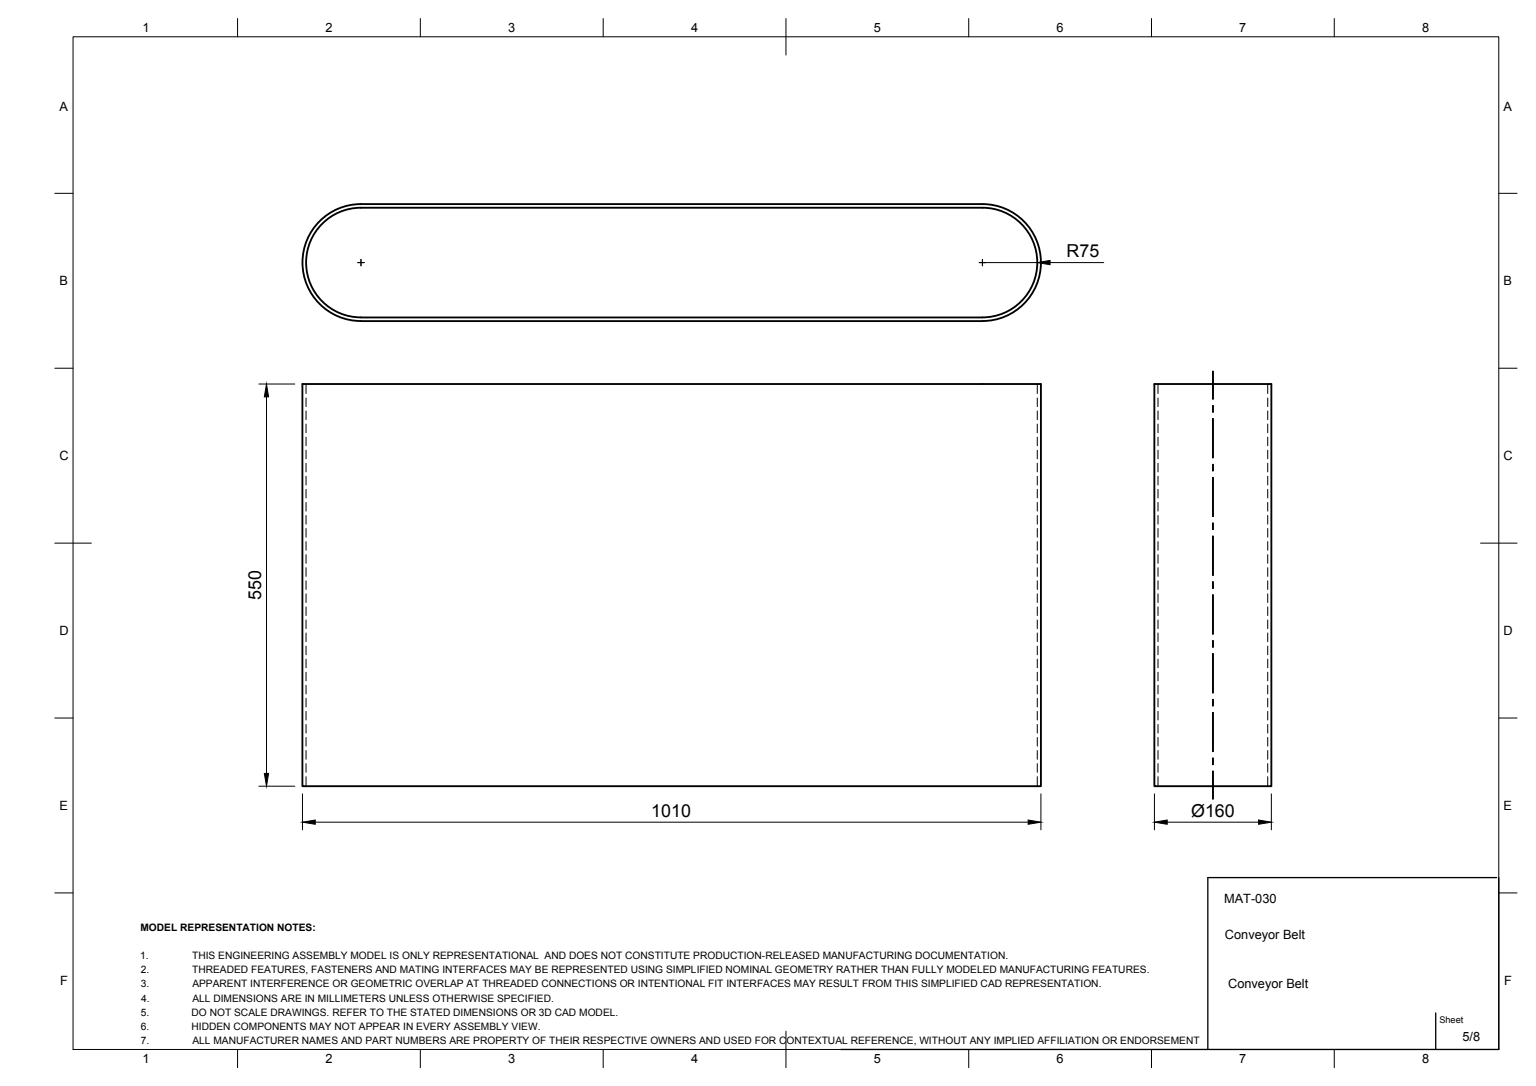
ISO-10303-21;
HEADER;
/* Generated by software containing ST-Developer
 * from STEP Tools, Inc. (www.steptools.com) 
 */

FILE_DESCRIPTION(
/* description */ ('STEP AP214'),
/* implementation_level */ '2;1');

FILE_NAME(
/* name */ 'Conveyor Belt.step',
/* time_stamp */ '2026-11-14T06:43:04-08:00',
/* author */ (''),
/* organization */ (''),
/* preprocessor_version */ 'ST-DEVELOPER v20.2',
/* originating_system */ 'Autodesk Translation Framework v15.17.0.0',
/* authorisation */ '');

FILE_SCHEMA (('AUTOMOTIVE_DESIGN { 1 0 10303 214 3 1 1 }'));
ENDSEC;

DATA;
#10=MECHANICAL_DESIGN_GEOMETRIC_PRESENTATION_REPRESENTATION('',(#198),#5658);
#176=SHAPE_REPRESENTATION_RELATIONSHIP('SRR','None',#5706,#187);
#187=ADVANCED_BREP_SHAPE_REPRESENTATION('',(#209),#5647);
#198=STYLED_ITEM('',(#5770),#209);
#209=MANIFOLD_SOLID_BREP('Body1',#3060);
#220=CYLINDRICAL_SURFACE('',#3205,80.);
#221=CYLINDRICAL_SURFACE('',#3207,80.);
#222=CYLINDRICAL_SURFACE('',#3209,75.);
#223=CYLINDRICAL_SURFACE('',#3211,75.);
#271=FACE_BOUND('',#520,.T.);
#272=FACE_BOUND('',#522,.T.);
#337=FACE_OUTER_BOUND('',#519,.T.);
#338=FACE_OUTER_BOUND('',#521,.T.);
#339=FACE_OUTER_BOUND('',#523,.T.);
#340=FACE_OUTER_BOUND('',#524,.T.);
#341=FACE_OUTER_BOUND('',#525,.T.);
#342=FACE_OUTER_BOUND('',#526,.T.);
#343=FACE_OUTER_BOUND('',#527,.T.);
#344=FACE_OUTER_BOUND('',#528,.T.);
#345=FACE_OUTER_BOUND('',#529,.T.);
#346=FACE_OUTER_BOUND('',#530,.T.);
#519=EDGE_LOOP('',(#1976,#1977,#1978,#1979));
#520=EDGE_LOOP('',(#1980,#1981,#1982,#1983));
#521=EDGE_LOOP('',(#1984,#1985,#1986,#1987));
#522=EDGE_LOOP('',(#1988,#1989,#1990,#1991));
#523=EDGE_LOOP('',(#1992,#1993,#1994,#1995));
#524=EDGE_LOOP('',(#1996,#1997,#1998,#1999));
#525=EDGE_LOOP('',(#2000,#2001,#2002,#2003));
#526=EDGE_LOOP('',(#2004,#2005,#2006,#2007));
#527=EDGE_LOOP('',(#2008,#2009,#2010,#2011));
#528=EDGE_LOOP('',(#2012,#2013,#2014,#2015));
#529=EDGE_LOOP('',(#2016,#2017,#2018,#2019));
#530=EDGE_LOOP('',(#2020,#2021,#2022,#2023));
#767=LINE('',#4494,#963);
#768=LINE('',#4497,#964);
#769=LINE('',#4500,#965);
#770=LINE('',#4504,#966);
#771=LINE('',#4511,#967);
#772=LINE('',#4514,#968);
#773=LINE('',#4519,#969);
#774=LINE('',#4522,#970);
#775=LINE('',#4524,#971);
#776=LINE('',#4525,#972);
#777=LINE('',#4527,#973);
#778=LINE('',#4529,#974);
#779=LINE('',#4532,#975);
#780=LINE('',#4533,#976);
#781=LINE('',#4535,#977);
#782=LINE('',#4537,#978);
#963=VECTOR('',#3567,1000.);
#964=VECTOR('',#3570,1000.);
#965=VECTOR('',#3571,1000.);
#966=VECTOR('',#3574,1000.);
#967=VECTOR('',#3581,1000.);
#968=VECTOR('',#3584,1000.);
#969=VECTOR('',#3587,1000.);
#970=VECTOR('',#3590,1000.);
#971=VECTOR('',#3593,1000.);
#972=VECTOR('',#3594,1000.);
#973=VECTOR('',#3597,1000.);
#974=VECTOR('',#3600,1000.);
#975=VECTOR('',#3605,1000.);
#976=VECTOR('',#3606,1000.);
#977=VECTOR('',#3609,1000.);
#978=VECTOR('',#3612,1000.);
#1159=CIRCLE('',#3196,80.);
#1160=CIRCLE('',#3197,80.);
#1161=CIRCLE('',#3198,75.);
#1162=CIRCLE('',#3199,75.);
#1163=CIRCLE('',#3201,80.);
#1164=CIRCLE('',#3202,80.);
#1165=CIRCLE('',#3203,75.);
#1166=CIRCLE('',#3204,75.);
#1314=VERTEX_POINT('',#4490);
#1315=VERTEX_POINT('',#4491);
#1316=VERTEX_POINT('',#4493);
#1317=VERTEX_POINT('',#4495);
#1318=VERTEX_POINT('',#4498);
#1319=VERTEX_POINT('',#4499);
#1320=VERTEX_POINT('',#4501);
#1321=VERTEX_POINT('',#4503);
#1322=VERTEX_POINT('',#4507);
#1323=VERTEX_POINT('',#4508);
#1324=VERTEX_POINT('',#4510);
#1325=VERTEX_POINT('',#4512);
#1326=VERTEX_POINT('',#4515);
#1327=VERTEX_POINT('',#4516);
#1328=VERTEX_POINT('',#4518);
#1329=VERTEX_POINT('',#4520);
#1571=EDGE_CURVE('',#1314,#1315,#1159,.T.);
#1572=EDGE_CURVE('',#1315,#1316,#767,.T.);
#1573=EDGE_CURVE('',#1316,#1317,#1160,.T.);
#1574=EDGE_CURVE('',#1317,#1314,#768,.T.);
#1575=EDGE_CURVE('',#1318,#1319,#769,.T.);
#1576=EDGE_CURVE('',#1320,#1318,#1161,.T.);
#1577=EDGE_CURVE('',#1321,#1320,#770,.T.);
#1578=EDGE_CURVE('',#1319,#1321,#1162,.T.);
#1579=EDGE_CURVE('',#1322,#1323,#1163,.T.);
#1580=EDGE_CURVE('',#1324,#1322,#771,.T.);
#1581=EDGE_CURVE('',#1325,#1324,#1164,.T.);
#1582=EDGE_CURVE('',#1323,#1325,#772,.T.);
#1583=EDGE_CURVE('',#1326,#1327,#1165,.T.);
#1584=EDGE_CURVE('',#1327,#1328,#773,.T.);
#1585=EDGE_CURVE('',#1328,#1329,#1166,.T.);
#1586=EDGE_CURVE('',#1329,#1326,#774,.T.);
#1587=EDGE_CURVE('',#1315,#1323,#775,.T.);
#1588=EDGE_CURVE('',#1314,#1322,#776,.T.);
#1589=EDGE_CURVE('',#1316,#1325,#777,.T.);
#1590=EDGE_CURVE('',#1317,#1324,#778,.T.);
#1591=EDGE_CURVE('',#1320,#1326,#779,.T.);
#1592=EDGE_CURVE('',#1318,#1327,#780,.T.);
#1593=EDGE_CURVE('',#1319,#1328,#781,.T.);
#1594=EDGE_CURVE('',#1321,#1329,#782,.T.);
#1976=ORIENTED_EDGE('',*,*,#1571,.T.);
#1977=ORIENTED_EDGE('',*,*,#1572,.T.);
#1978=ORIENTED_EDGE('',*,*,#1573,.T.);
#1979=ORIENTED_EDGE('',*,*,#1574,.T.);
#1980=ORIENTED_EDGE('',*,*,#1575,.F.);
#1981=ORIENTED_EDGE('',*,*,#1576,.F.);
#1982=ORIENTED_EDGE('',*,*,#1577,.F.);
#1983=ORIENTED_EDGE('',*,*,#1578,.F.);
#1984=ORIENTED_EDGE('',*,*,#1579,.F.);
#1985=ORIENTED_EDGE('',*,*,#1580,.F.);
#1986=ORIENTED_EDGE('',*,*,#1581,.F.);
#1987=ORIENTED_EDGE('',*,*,#1582,.F.);
#1988=ORIENTED_EDGE('',*,*,#1583,.T.);
#1989=ORIENTED_EDGE('',*,*,#1584,.T.);
#1990=ORIENTED_EDGE('',*,*,#1585,.T.);
#1991=ORIENTED_EDGE('',*,*,#1586,.T.);
#1992=ORIENTED_EDGE('',*,*,#1579,.T.);
#1993=ORIENTED_EDGE('',*,*,#1587,.F.);
#1994=ORIENTED_EDGE('',*,*,#1571,.F.);
#1995=ORIENTED_EDGE('',*,*,#1588,.T.);
#1996=ORIENTED_EDGE('',*,*,#1582,.T.);
#1997=ORIENTED_EDGE('',*,*,#1589,.F.);
#1998=ORIENTED_EDGE('',*,*,#1572,.F.);
#1999=ORIENTED_EDGE('',*,*,#1587,.T.);
#2000=ORIENTED_EDGE('',*,*,#1581,.T.);
#2001=ORIENTED_EDGE('',*,*,#1590,.F.);
#2002=ORIENTED_EDGE('',*,*,#1573,.F.);
#2003=ORIENTED_EDGE('',*,*,#1589,.T.);
#2004=ORIENTED_EDGE('',*,*,#1580,.T.);
#2005=ORIENTED_EDGE('',*,*,#1588,.F.);
#2006=ORIENTED_EDGE('',*,*,#1574,.F.);
#2007=ORIENTED_EDGE('',*,*,#1590,.T.);
#2008=ORIENTED_EDGE('',*,*,#1583,.F.);
#2009=ORIENTED_EDGE('',*,*,#1591,.F.);
#2010=ORIENTED_EDGE('',*,*,#1576,.T.);
#2011=ORIENTED_EDGE('',*,*,#1592,.T.);
#2012=ORIENTED_EDGE('',*,*,#1584,.F.);
#2013=ORIENTED_EDGE('',*,*,#1592,.F.);
#2014=ORIENTED_EDGE('',*,*,#1575,.T.);
#2015=ORIENTED_EDGE('',*,*,#1593,.T.);
#2016=ORIENTED_EDGE('',*,*,#1585,.F.);
#2017=ORIENTED_EDGE('',*,*,#1593,.F.);
#2018=ORIENTED_EDGE('',*,*,#1578,.T.);
#2019=ORIENTED_EDGE('',*,*,#1594,.T.);
#2020=ORIENTED_EDGE('',*,*,#1586,.F.);
#2021=ORIENTED_EDGE('',*,*,#1594,.F.);
#2022=ORIENTED_EDGE('',*,*,#1577,.T.);
#2023=ORIENTED_EDGE('',*,*,#1591,.T.);
#2786=PLANE('',#3195);
#2787=PLANE('',#3200);
#2788=PLANE('',#3206);
#2789=PLANE('',#3208);
#2790=PLANE('',#3210);
#2791=PLANE('',#3212);
#2878=ADVANCED_FACE('',(#337,#271),#2786,.T.);
#2879=ADVANCED_FACE('',(#338,#272),#2787,.F.);
#2880=ADVANCED_FACE('',(#339),#220,.T.);
#2881=ADVANCED_FACE('',(#340),#2788,.F.);
#2882=ADVANCED_FACE('',(#341),#221,.T.);
#2883=ADVANCED_FACE('',(#342),#2789,.F.);
#2884=ADVANCED_FACE('',(#343),#222,.F.);
#2885=ADVANCED_FACE('',(#344),#2790,.T.);
#2886=ADVANCED_FACE('',(#345),#223,.F.);
#2887=ADVANCED_FACE('',(#346),#2791,.T.);
#3060=CLOSED_SHELL('',(#2878,#2879,#2880,#2881,#2882,#2883,#2884,#2885,
#2886,#2887));
#3194=AXIS2_PLACEMENT_3D('',#4488,#3561,#3562);
#3195=AXIS2_PLACEMENT_3D('',#4489,#3563,#3564);
#3196=AXIS2_PLACEMENT_3D('',#4492,#3565,#3566);
#3197=AXIS2_PLACEMENT_3D('',#4496,#3568,#3569);
#3198=AXIS2_PLACEMENT_3D('',#4502,#3572,#3573);
#3199=AXIS2_PLACEMENT_3D('',#4505,#3575,#3576);
#3200=AXIS2_PLACEMENT_3D('',#4506,#3577,#3578);
#3201=AXIS2_PLACEMENT_3D('',#4509,#3579,#3580);
#3202=AXIS2_PLACEMENT_3D('',#4513,#3582,#3583);
#3203=AXIS2_PLACEMENT_3D('',#4517,#3585,#3586);
#3204=AXIS2_PLACEMENT_3D('',#4521,#3588,#3589);
#3205=AXIS2_PLACEMENT_3D('',#4523,#3591,#3592);
#3206=AXIS2_PLACEMENT_3D('',#4526,#3595,#3596);
#3207=AXIS2_PLACEMENT_3D('',#4528,#3598,#3599);
#3208=AXIS2_PLACEMENT_3D('',#4530,#3601,#3602);
#3209=AXIS2_PLACEMENT_3D('',#4531,#3603,#3604);
#3210=AXIS2_PLACEMENT_3D('',#4534,#3607,#3608);
#3211=AXIS2_PLACEMENT_3D('',#4536,#3610,#3611);
#3212=AXIS2_PLACEMENT_3D('',#4538,#3613,#3614);
#3561=DIRECTION('axis',(0.,0.,1.));
#3562=DIRECTION('refdir',(1.,0.,0.));
#3563=DIRECTION('center_axis',(1.,0.,0.));
#3564=DIRECTION('ref_axis',(0.,0.,-1.));
#3565=DIRECTION('center_axis',(1.,0.,0.));
#3566=DIRECTION('ref_axis',(0.,1.,0.));
#3567=DIRECTION('',(0.,1.,1.79594901042305E-16));
#3568=DIRECTION('center_axis',(1.,0.,0.));
#3569=DIRECTION('ref_axis',(0.,1.,0.));
#3570=DIRECTION('',(0.,-1.,-1.79594901042305E-16));
#3571=DIRECTION('',(0.,1.,1.79594901042305E-16));
#3572=DIRECTION('center_axis',(1.,0.,0.));
#3573=DIRECTION('ref_axis',(0.,0.,-1.));
#3574=DIRECTION('',(0.,-1.,-1.79594901042305E-16));
#3575=DIRECTION('center_axis',(1.,0.,0.));
#3576=DIRECTION('ref_axis',(0.,0.,-1.));
#3577=DIRECTION('center_axis',(1.,0.,0.));
#3578=DIRECTION('ref_axis',(0.,0.,-1.));
#3579=DIRECTION('center_axis',(1.,0.,0.));
#3580=DIRECTION('ref_axis',(0.,1.,0.));
#3581=DIRECTION('',(0.,-1.,-1.79594901042305E-16));
#3582=DIRECTION('center_axis',(1.,0.,0.));
#3583=DIRECTION('ref_axis',(0.,1.,0.));
#3584=DIRECTION('',(0.,1.,1.79594901042305E-16));
#3585=DIRECTION('center_axis',(1.,0.,0.));
#3586=DIRECTION('ref_axis',(0.,0.,-1.));
#3587=DIRECTION('',(0.,1.,1.79594901042305E-16));
#3588=DIRECTION('center_axis',(1.,0.,0.));
#3589=DIRECTION('ref_axis',(0.,0.,-1.));
#3590=DIRECTION('',(0.,-1.,-1.79594901042305E-16));
#3591=DIRECTION('center_axis',(-1.,0.,0.));
#3592=DIRECTION('ref_axis',(0.,0.,1.));
#3593=DIRECTION('',(-1.,0.,0.));
#3594=DIRECTION('',(-1.,0.,0.));
#3595=DIRECTION('center_axis',(0.,-1.79594901042305E-16,1.));
#3596=DIRECTION('ref_axis',(0.,-1.,-1.79594901042305E-16));
#3597=DIRECTION('',(-1.,0.,0.));
#3598=DIRECTION('center_axis',(-1.,0.,0.));
#3599=DIRECTION('ref_axis',(0.,0.,1.));
#3600=DIRECTION('',(-1.,0.,0.));
#3601=DIRECTION('center_axis',(0.,1.79594901042305E-16,-1.));
#3602=DIRECTION('ref_axis',(0.,1.,1.79594901042305E-16));
#3603=DIRECTION('center_axis',(-1.,0.,0.));
#3604=DIRECTION('ref_axis',(0.,0.,1.));
#3605=DIRECTION('',(-1.,0.,0.));
#3606=DIRECTION('',(-1.,0.,0.));
#3607=DIRECTION('center_axis',(0.,-1.79594901042305E-16,1.));
#3608=DIRECTION('ref_axis',(0.,-1.,-1.79594901042305E-16));
#3609=DIRECTION('',(-1.,0.,0.));
#3610=DIRECTION('center_axis',(-1.,0.,0.));
#3611=DIRECTION('ref_axis',(0.,0.,1.));
#3612=DIRECTION('',(-1.,0.,0.));
#3613=DIRECTION('center_axis',(0.,1.79594901042305E-16,-1.));
#3614=DIRECTION('ref_axis',(0.,1.,1.79594901042305E-16));
#4488=CARTESIAN_POINT('',(0.,0.,0.));
#4489=CARTESIAN_POINT('Origin',(275.,-425.,0.));
#4490=CARTESIAN_POINT('',(275.,-425.,80.));
#4491=CARTESIAN_POINT('',(275.,-425.,-80.));
#4492=CARTESIAN_POINT('Origin',(275.,-425.,0.));
#4493=CARTESIAN_POINT('',(275.,425.,-79.9999999999998));
#4494=CARTESIAN_POINT('',(275.,-425.,-80.));
#4495=CARTESIAN_POINT('',(275.,425.,80.0000000000002));
#4496=CARTESIAN_POINT('Origin',(275.,425.,1.56142466891288E-13));
#4497=CARTESIAN_POINT('',(275.,-425.,80.));
#4498=CARTESIAN_POINT('',(275.,-425.,-75.));
#4499=CARTESIAN_POINT('',(275.,425.,-74.9999999999998));
#4500=CARTESIAN_POINT('',(275.,-425.,-75.));
#4501=CARTESIAN_POINT('',(275.,-425.,75.));
#4502=CARTESIAN_POINT('Origin',(275.,-425.,0.));
#4503=CARTESIAN_POINT('',(275.,425.,75.0000000000002));
#4504=CARTESIAN_POINT('',(275.,-425.,75.));
#4505=CARTESIAN_POINT('Origin',(275.,425.,1.56142466891288E-13));
#4506=CARTESIAN_POINT('Origin',(-275.,-425.,0.));
#4507=CARTESIAN_POINT('',(-275.,-425.,80.));
#4508=CARTESIAN_POINT('',(-275.,-425.,-80.));
#4509=CARTESIAN_POINT('Origin',(-275.,-425.,0.));
#4510=CARTESIAN_POINT('',(-275.,425.,80.0000000000002));
#4511=CARTESIAN_POINT('',(-275.,-425.,80.));
#4512=CARTESIAN_POINT('',(-275.,425.,-79.9999999999998));
#4513=CARTESIAN_POINT('Origin',(-275.,425.,1.56142466891288E-13));
#4514=CARTESIAN_POINT('',(-275.,-425.,-80.));
#4515=CARTESIAN_POINT('',(-275.,-425.,75.));
#4516=CARTESIAN_POINT('',(-275.,-425.,-75.));
#4517=CARTESIAN_POINT('Origin',(-275.,-425.,0.));
#4518=CARTESIAN_POINT('',(-275.,425.,-74.9999999999998));
#4519=CARTESIAN_POINT('',(-275.,-425.,-75.));
#4520=CARTESIAN_POINT('',(-275.,425.,75.0000000000002));
#4521=CARTESIAN_POINT('Origin',(-275.,425.,1.56142466891288E-13));
#4522=CARTESIAN_POINT('',(-275.,-425.,75.));
#4523=CARTESIAN_POINT('Origin',(275.,-425.,0.));
#4524=CARTESIAN_POINT('',(275.,-425.,-80.));
#4525=CARTESIAN_POINT('',(275.,-425.,80.));
#4526=CARTESIAN_POINT('Origin',(275.,-425.,-80.));
#4527=CARTESIAN_POINT('',(275.,425.,-79.9999999999998));
#4528=CARTESIAN_POINT('Origin',(275.,425.,1.56142466891288E-13));
#4529=CARTESIAN_POINT('',(275.,425.,80.0000000000002));
#4530=CARTESIAN_POINT('Origin',(275.,-425.,80.));
#4531=CARTESIAN_POINT('Origin',(275.,-425.,0.));
#4532=CARTESIAN_POINT('',(275.,-425.,75.));
#4533=CARTESIAN_POINT('',(275.,-425.,-75.));
#4534=CARTESIAN_POINT('Origin',(275.,-425.,-75.));
#4535=CARTESIAN_POINT('',(275.,425.,-74.9999999999998));
#4536=CARTESIAN_POINT('Origin',(275.,425.,1.56142466891288E-13));
#4537=CARTESIAN_POINT('',(275.,425.,75.0000000000002));
#4538=CARTESIAN_POINT('Origin',(275.,-425.,75.));
#5634=UNCERTAINTY_MEASURE_WITH_UNIT(LENGTH_MEASURE(0.01),#5659,
'DISTANCE_ACCURACY_VALUE',
'Maximum model space distance between geometric entities at asserted c
onnectivities');
#5645=UNCERTAINTY_MEASURE_WITH_UNIT(LENGTH_MEASURE(0.01),#5659,
'DISTANCE_ACCURACY_VALUE',
'Maximum model space distance between geometric entities at asserted c
onnectivities');
#5647=(
GEOMETRIC_REPRESENTATION_CONTEXT(3)
GLOBAL_UNCERTAINTY_ASSIGNED_CONTEXT((#5634))
GLOBAL_UNIT_ASSIGNED_CONTEXT((#5659,#5661,#5662))
REPRESENTATION_CONTEXT('','3D')
);
#5658=(
GEOMETRIC_REPRESENTATION_CONTEXT(3)
GLOBAL_UNCERTAINTY_ASSIGNED_CONTEXT((#5645))
GLOBAL_UNIT_ASSIGNED_CONTEXT((#5659,#5661,#5662))
REPRESENTATION_CONTEXT('','3D')
);
#5659=(
LENGTH_UNIT()
NAMED_UNIT(*)
SI_UNIT(.MILLI.,.METRE.)
);
#5661=(
NAMED_UNIT(*)
PLANE_ANGLE_UNIT()
SI_UNIT($,.RADIAN.)
);
#5662=(
NAMED_UNIT(*)
SI_UNIT($,.STERADIAN.)
SOLID_ANGLE_UNIT()
);
#5664=SHAPE_DEFINITION_REPRESENTATION(#5676,#5706);
#5676=PRODUCT_DEFINITION_SHAPE('',$,#5719);
#5706=SHAPE_REPRESENTATION('',(#3194),#5647);
#5717=PRODUCT_DEFINITION_CONTEXT('part definition',#5755,'design');
#5719=PRODUCT_DEFINITION('Conveyor Belt','Conveyor Belt',#5731,#5717);
#5731=PRODUCT_DEFINITION_FORMATION('',$,#5758);
#5755=APPLICATION_CONTEXT(
'Core Data for Automotive Mechanical Design Process');
#5756=PRODUCT_CONTEXT('part definition',#5755,'mechanical');
#5758=PRODUCT('Conveyor Belt','Conveyor Belt',$,(#5756));
#5770=PRESENTATION_STYLE_ASSIGNMENT((#5775));
#5775=SURFACE_STYLE_USAGE(.BOTH.,#5780);
#5780=SURFACE_SIDE_STYLE('',(#5785));
#5785=SURFACE_STYLE_FILL_AREA(#5790);
#5790=FILL_AREA_STYLE('Opaque(31,36,43)',(#5795));
#5795=FILL_AREA_STYLE_COLOUR('Opaque(31,36,43)',#5800);
#5800=COLOUR_RGB('Opaque(31,36,43)',0.12156862745098,0.141176470588235,
0.168627450980392);
ENDSEC;
END-ISO-10303-21;
